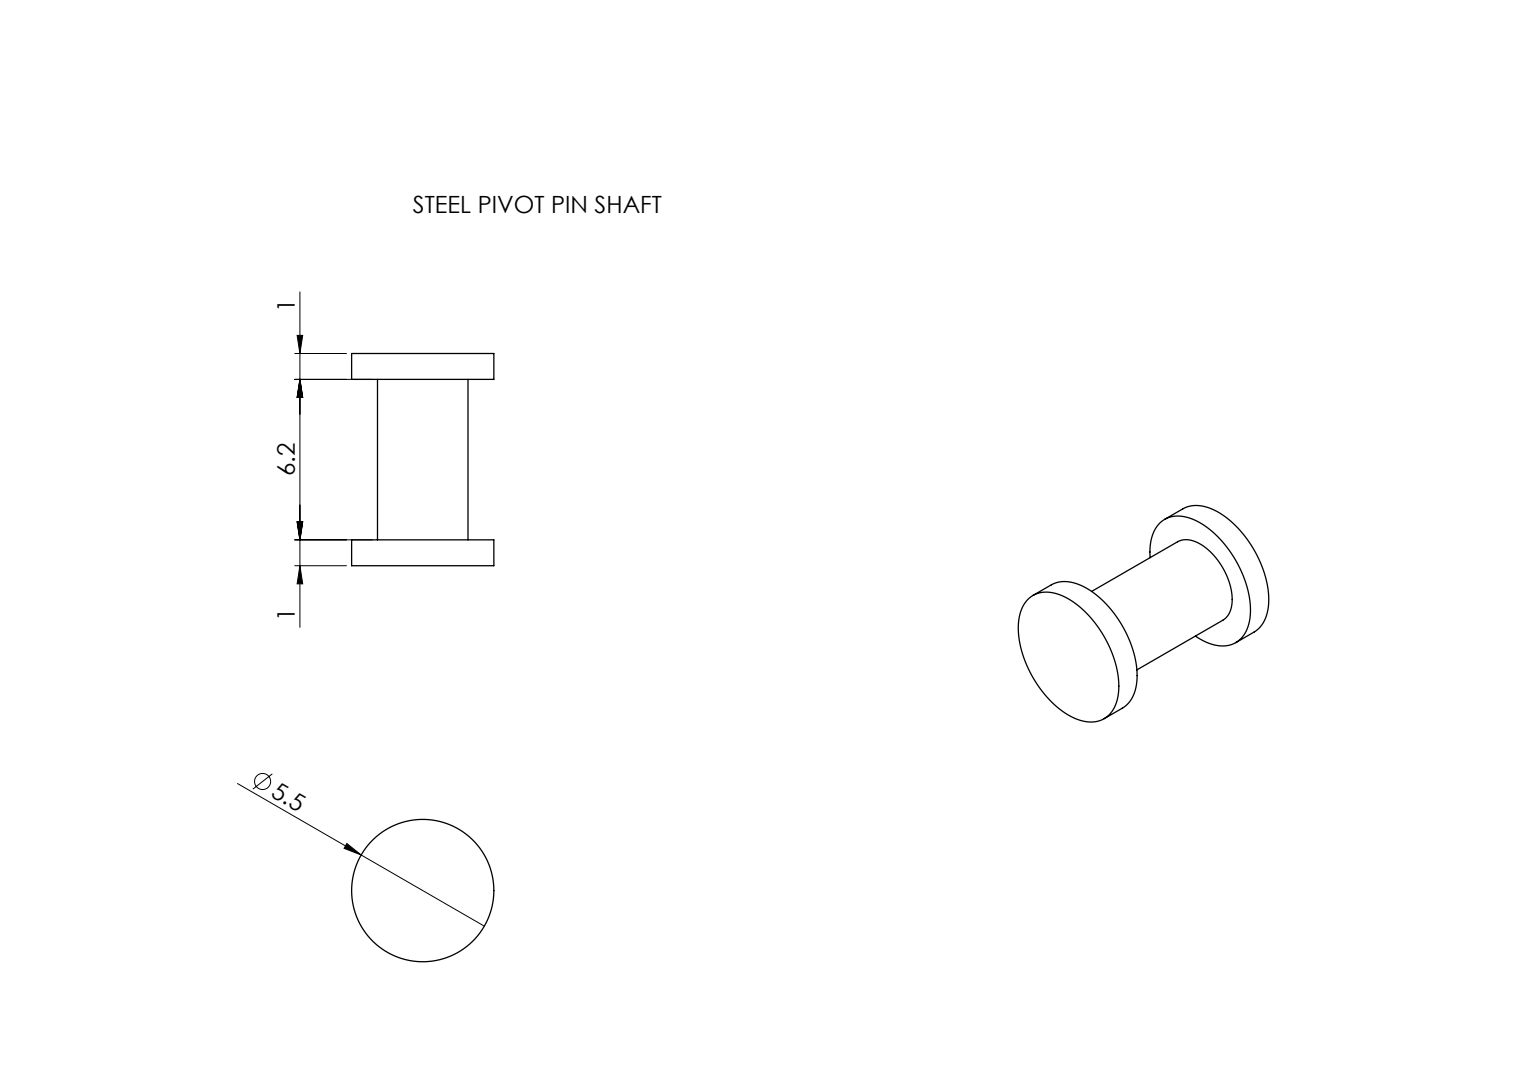
ISO-10303-21;
HEADER;
FILE_DESCRIPTION (('STEP AP214'),
    '1' );
FILE_NAME ('Steel Pivot Pin Shaft.step',
    '2026-09-30T04:43:20',
    ( '' ),
    ( '' ),
    'SwSTEP 2.0',
    'SolidWorks 2026',
    '' );
FILE_SCHEMA (( 'AUTOMOTIVE_DESIGN' ));
ENDSEC;

DATA;
#339=EDGE_CURVE ( 'NONE', #23586, #15428, #53300, .T. ) ;
#351=CARTESIAN_POINT ( 'NONE',  ( -6.110905869600904872, 1.712176620043476140E-14, 3.600000000000000089 ) ) ;
#366=EDGE_LOOP ( 'NONE', ( #1218, #51641 ) ) ;
#396=ORIENTED_EDGE ( 'NONE', *, *, #51721, .F. ) ;
#484=DIRECTION ( 'NONE',  ( 0.000000000000000000, 0.000000000000000000, 1.000000000000000000 ) ) ;
#1065=DIRECTION ( 'NONE',  ( 0.000000000000000000, 0.000000000000000000, -1.000000000000000000 ) ) ;
#1143=ORIENTED_EDGE ( 'NONE', *, *, #9429, .T. ) ;
#1218=ORIENTED_EDGE ( 'NONE', *, *, #16405, .T. ) ;
#1370=EDGE_LOOP ( 'NONE', ( #41531, #53817 ) ) ;
#1691=AXIS2_PLACEMENT_3D ( 'NONE', #351, #44090, #52871 ) ;
#1703=CARTESIAN_POINT ( 'NONE',  ( -6.110905869600904872, 1.712176620043476140E-14, -3.600000000000000089 ) ) ;
#1760=( GEOMETRIC_REPRESENTATION_CONTEXT ( 3 ) GLOBAL_UNCERTAINTY_ASSIGNED_CONTEXT ( ( #42179 ) ) GLOBAL_UNIT_ASSIGNED_CONTEXT ( ( #39762, #23813, #2772 ) ) REPRESENTATION_CONTEXT ( 'NONE', 'WORKASPACE' ) );
#1875=VERTEX_POINT ( 'NONE', #20074 ) ;
#1894=EDGE_LOOP ( 'NONE', ( #21734, #23060 ) ) ;
#2067=EDGE_LOOP ( 'NONE', ( #37855, #52540, #10327, #27541 ) ) ;
#2068=DIRECTION ( 'NONE',  ( -1.000000000000000000, 0.000000000000000000, 0.000000000000000000 ) ) ;
#2078=AXIS2_PLACEMENT_3D ( 'NONE', #1703, #6268, #15329 ) ;
#2169=EDGE_CURVE ( 'NONE', #13325, #33916, #33726, .T. ) ;
#2253=VECTOR ( 'NONE', #43903, 1000.000000000000000 ) ;
#2401=CARTESIAN_POINT ( 'NONE',  ( -6.110905869600904872, 1.712176620043476140E-14, 2.600000000000000089 ) ) ;
#2458=FACE_OUTER_BOUND ( 'NONE', #1370, .T. ) ;
#2610=AXIS2_PLACEMENT_3D ( 'NONE', #34638, #13373, #3697 ) ;
#2772=( NAMED_UNIT ( * ) SI_UNIT ( $, .STERADIAN. ) SOLID_ANGLE_UNIT ( ) );
#3052=CARTESIAN_POINT ( 'NONE',  ( -3.360905869600907092, 1.745854407020028306E-14, 3.600000000000000089 ) ) ;
#3156=SHAPE_REPRESENTATION ( 'Steel Pivot Pin Shaft', ( #2610 ), #1760 ) ;
#3558=UNCERTAINTY_MEASURE_WITH_UNIT (LENGTH_MEASURE( 1.000000000000000082E-05 ), #11031, 'distance_accuracy_value', 'NONE');
#3697=DIRECTION ( 'NONE',  ( 1.000000000000000000, 0.000000000000000000, 0.000000000000000000 ) ) ;
#3719=ADVANCED_FACE ( 'NONE', ( #23132 ), #6367, .T. ) ;
#4027=AXIS2_PLACEMENT_3D ( 'NONE', #41047, #46142, #45878 ) ;
#4059=CIRCLE ( 'NONE', #6771, 2.749999999999997335 ) ;
#4638=DIRECTION ( 'NONE',  ( -1.000000000000000000, 0.000000000000000000, 0.000000000000000000 ) ) ;
#5017=ORIENTED_EDGE ( 'NONE', *, *, #54598, .F. ) ;
#5743=APPLICATION_CONTEXT ( 'automotive_design' ) ;
#5928=AXIS2_PLACEMENT_3D ( 'NONE', #44296, #53097, #40307 ) ;
#6268=DIRECTION ( 'NONE',  ( 0.000000000000000000, 0.000000000000000000, -1.000000000000000000 ) ) ;
#6367=CYLINDRICAL_SURFACE ( 'NONE', #37649, 1.750000000000003331 ) ;
#6536=AXIS2_PLACEMENT_3D ( 'NONE', #26903, #484, #8748 ) ;
#6615=VERTEX_POINT ( 'NONE', #41477 ) ;
#6732=EDGE_CURVE ( 'NONE', #6615, #10587, #21831, .T. ) ;
#6771=AXIS2_PLACEMENT_3D ( 'NONE', #23374, #27624, #40690 ) ;
#6831=CLOSED_SHELL ( 'NONE', ( #47988, #39827, #3719, #23415, #26829, #43131, #39539, #24833, #28152, #23876 ) ) ;
#6962=DIRECTION ( 'NONE',  ( 0.000000000000000000, 0.000000000000000000, 1.000000000000000000 ) ) ;
#6987=VERTEX_POINT ( 'NONE', #32867 ) ;
#7083=FILL_AREA_STYLE_COLOUR ( '', #10850 ) ;
#7134=CARTESIAN_POINT ( 'NONE',  ( -3.360905869600907092, 1.712176620043476140E-14, -3.600000000000000089 ) ) ;
#7765=CARTESIAN_POINT ( 'NONE',  ( -8.860905869600903983, 1.712176620043476140E-14, 3.600000000000000089 ) ) ;
#7964=DIRECTION ( 'NONE',  ( -0.000000000000000000, -0.000000000000000000, 1.000000000000000000 ) ) ;
#8573=VECTOR ( 'NONE', #42169, 1000.000000000000000 ) ;
#8748=DIRECTION ( 'NONE',  ( 1.000000000000000000, 0.000000000000000000, 0.000000000000000000 ) ) ;
#9041=CARTESIAN_POINT ( 'NONE',  ( -4.360905869600901319, 1.733607939028554791E-14, -3.600000000000000089 ) ) ;
#9135=ORIENTED_EDGE ( 'NONE', *, *, #55863, .F. ) ;
#9429=EDGE_CURVE ( 'NONE', #6987, #33042, #15488, .T. ) ;
#9446=CARTESIAN_POINT ( 'NONE',  ( -6.110905869600904872, 1.712176620043476140E-14, 2.600000000000000089 ) ) ;
#9702=CYLINDRICAL_SURFACE ( 'NONE', #40281, 2.749999999999997780 ) ;
#9786=ORIENTED_EDGE ( 'NONE', *, *, #25713, .F. ) ;
#10212=AXIS2_PLACEMENT_3D ( 'NONE', #50763, #55050, #45962 ) ;
#10236=DIRECTION ( 'NONE',  ( 1.000000000000000000, 0.000000000000000000, 0.000000000000000000 ) ) ;
#10327=ORIENTED_EDGE ( 'NONE', *, *, #54598, .T. ) ;
#10570=FILL_AREA_STYLE_COLOUR ( '', #28482 ) ;
#10587=VERTEX_POINT ( 'NONE', #20963 ) ;
#10850=COLOUR_RGB ( '', 0.72549020, 0.75294118, 0.79215686) ;
#11031=( LENGTH_UNIT ( ) NAMED_UNIT ( * ) SI_UNIT ( .MILLI., .METRE. ) );
#11661=FILL_AREA_STYLE ('',( #10570 ) ) ;
#11865=SURFACE_STYLE_USAGE ( .BOTH. , #32620 ) ;
#12149=MECHANICAL_DESIGN_GEOMETRIC_PRESENTATION_REPRESENTATION('',(#43002),#55684);
#12473=DIRECTION ( 'NONE',  ( 0.000000000000000000, 0.000000000000000000, 1.000000000000000000 ) ) ;
#12683=MECHANICAL_DESIGN_GEOMETRIC_PRESENTATION_REPRESENTATION('',(#46182),#19000);
#13325=VERTEX_POINT ( 'NONE', #15566 ) ;
#13373=DIRECTION ( 'NONE',  ( 0.000000000000000000, 0.000000000000000000, 1.000000000000000000 ) ) ;
#13649=DIRECTION ( 'NONE',  ( -0.000000000000000000, -0.000000000000000000, 1.000000000000000000 ) ) ;
#13919=ORIENTED_EDGE ( 'NONE', *, *, #51721, .T. ) ;
#14396=CARTESIAN_POINT ( 'NONE',  ( -3.360905869600907092, 1.712176620043476140E-14, -4.599999999999999645 ) ) ;
#14547=DIRECTION ( 'NONE',  ( 0.000000000000000000, 0.000000000000000000, 1.000000000000000000 ) ) ;
#14842=AXIS2_PLACEMENT_3D ( 'NONE', #40048, #27012, #10236 ) ;
#14859=EDGE_LOOP ( 'NONE', ( #20763, #21521, #39292, #31255 ) ) ;
#15099=SURFACE_STYLE_USAGE ( .BOTH. , #45722 ) ;
#15329=DIRECTION ( 'NONE',  ( -1.000000000000000000, 0.000000000000000000, -0.000000000000000000 ) ) ;
#15428=VERTEX_POINT ( 'NONE', #7134 ) ;
#15488=CIRCLE ( 'NONE', #46317, 1.750000000000003331 ) ;
#15566=CARTESIAN_POINT ( 'NONE',  ( -8.860905869600903983, 1.712176620043476140E-14, 3.600000000000000089 ) ) ;
#16398=EDGE_CURVE ( 'NONE', #33916, #43669, #20608, .T. ) ;
#16405=EDGE_CURVE ( 'NONE', #53889, #44242, #24860, .T. ) ;
#16724=ORIENTED_EDGE ( 'NONE', *, *, #9429, .F. ) ;
#17002=EDGE_LOOP ( 'NONE', ( #45520, #34695 ) ) ;
#17694=PLANE ( 'NONE',  #33826 ) ;
#17939=FACE_OUTER_BOUND ( 'NONE', #14859, .T. ) ;
#18204=EDGE_CURVE ( 'NONE', #33042, #6987, #54958, .T. ) ;
#18215=CARTESIAN_POINT ( 'NONE',  ( -6.110905869600904872, 1.712176620043476140E-14, -3.600000000000000089 ) ) ;
#18260=PRODUCT_DEFINITION_SHAPE ( 'NONE', 'NONE',  #35061 ) ;
#18382=AXIS2_PLACEMENT_3D ( 'NONE', #24725, #33816, #29581 ) ;
#18499=AXIS2_PLACEMENT_3D ( 'NONE', #49858, #28274, #37345 ) ;
#18809=DIRECTION ( 'NONE',  ( 0.000000000000000000, 0.000000000000000000, 1.000000000000000000 ) ) ;
#19000=( GEOMETRIC_REPRESENTATION_CONTEXT ( 3 ) GLOBAL_UNCERTAINTY_ASSIGNED_CONTEXT ( ( #3558 ) ) GLOBAL_UNIT_ASSIGNED_CONTEXT ( ( #11031, #40863, #33466 ) ) REPRESENTATION_CONTEXT ( 'NONE', 'WORKASPACE' ) );
#19278=CARTESIAN_POINT ( 'NONE',  ( -4.360905869600901319, 1.733607939028554791E-14, 2.600000000000000089 ) ) ;
#19415=CARTESIAN_POINT ( 'NONE',  ( -4.360905869600901319, 1.733607939028554791E-14, 2.600000000000000089 ) ) ;
#19808=CIRCLE ( 'NONE', #1691, 2.749999999999998224 ) ;
#19916=PRODUCT_DEFINITION_FORMATION_WITH_SPECIFIED_SOURCE ( 'ANY', '', #27850, .NOT_KNOWN. ) ;
#20074=CARTESIAN_POINT ( 'NONE',  ( -8.860905869600903983, 1.712176620043476140E-14, 2.600000000000000089 ) ) ;
#20081=AXIS2_PLACEMENT_3D ( 'NONE', #48959, #44994, #2068 ) ;
#20150=PRESENTATION_STYLE_ASSIGNMENT (( #15099 ) ) ;
#20201=CIRCLE ( 'NONE', #10212, 2.749999999999998224 ) ;
#20608=LINE ( 'NONE', #28264, #8573 ) ;
#20695=SHAPE_DEFINITION_REPRESENTATION ( #18260, #3156 ) ;
#20763=ORIENTED_EDGE ( 'NONE', *, *, #6732, .F. ) ;
#20963=CARTESIAN_POINT ( 'NONE',  ( -8.860905869600902207, 1.745854407020028306E-14, -3.600000000000000089 ) ) ;
#21107=CARTESIAN_POINT ( 'NONE',  ( -6.110905869600904872, 1.712176620043476140E-14, -4.599999999999999645 ) ) ;
#21394=ORIENTED_EDGE ( 'NONE', *, *, #16405, .F. ) ;
#21478=EDGE_CURVE ( 'NONE', #1875, #43669, #20201, .T. ) ;
#21521=ORIENTED_EDGE ( 'NONE', *, *, #42925, .F. ) ;
#21734=ORIENTED_EDGE ( 'NONE', *, *, #2169, .T. ) ;
#21831=LINE ( 'NONE', #46855, #54507 ) ;
#21855=DIRECTION ( 'NONE',  ( -1.000000000000000000, 0.000000000000000000, 0.000000000000000000 ) ) ;
#22356=DIRECTION ( 'NONE',  ( -0.000000000000000000, -0.000000000000000000, 1.000000000000000000 ) ) ;
#22763=DIRECTION ( 'NONE',  ( 1.000000000000000000, 0.000000000000000000, 0.000000000000000000 ) ) ;
#23060=ORIENTED_EDGE ( 'NONE', *, *, #55863, .T. ) ;
#23072=FACE_OUTER_BOUND ( 'NONE', #17002, .T. ) ;
#23132=FACE_OUTER_BOUND ( 'NONE', #53242, .T. ) ;
#23250=DIRECTION ( 'NONE',  ( -1.000000000000000000, 0.000000000000000000, 0.000000000000000000 ) ) ;
#23374=CARTESIAN_POINT ( 'NONE',  ( -6.110905869600904872, 1.712176620043476140E-14, -3.600000000000000089 ) ) ;
#23415=ADVANCED_FACE ( 'NONE', ( #43809 ), #34738, .T. ) ;
#23458=ORIENTED_EDGE ( 'NONE', *, *, #6732, .T. ) ;
#23586=VERTEX_POINT ( 'NONE', #42905 ) ;
#23813=( NAMED_UNIT ( * ) PLANE_ANGLE_UNIT ( ) SI_UNIT ( $, .RADIAN. ) );
#23837=FACE_OUTER_BOUND ( 'NONE', #51240, .T. ) ;
#23876=ADVANCED_FACE ( 'NONE', ( #27550, #23837 ), #49947, .F. ) ;
#24166=AXIS2_PLACEMENT_3D ( 'NONE', #53600, #1065, #23250 ) ;
#24573=DIRECTION ( 'NONE',  ( 0.000000000000000000, 0.000000000000000000, -1.000000000000000000 ) ) ;
#24725=CARTESIAN_POINT ( 'NONE',  ( -6.110905869600904872, 1.712176620043476140E-14, 3.600000000000000089 ) ) ;
#24833=ADVANCED_FACE ( 'NONE', ( #17939 ), #9702, .T. ) ;
#24860=CIRCLE ( 'NONE', #4027, 1.750000000000003331 ) ;
#25713=EDGE_CURVE ( 'NONE', #53889, #6987, #43073, .T. ) ;
#26591=ADVANCED_BREP_SHAPE_REPRESENTATION ( '', ( #41703, #2610 ), #1760 ) ;
#26774=ORIENTED_EDGE ( 'NONE', *, *, #37370, .T. ) ;
#26829=ADVANCED_FACE ( 'NONE', ( #40983 ), #35923, .T. ) ;
#26903=CARTESIAN_POINT ( 'NONE',  ( -6.110905869600904872, 1.712176620043476140E-14, 3.600000000000000089 ) ) ;
#27012=DIRECTION ( 'NONE',  ( -0.000000000000000000, -0.000000000000000000, 1.000000000000000000 ) ) ;
#27541=ORIENTED_EDGE ( 'NONE', *, *, #21478, .T. ) ;
#27550=FACE_BOUND ( 'NONE', #39735, .T. ) ;
#27624=DIRECTION ( 'NONE',  ( 0.000000000000000000, 0.000000000000000000, -1.000000000000000000 ) ) ;
#27850=PRODUCT ( 'Steel Pivot Pin Shaft', 'Steel Pivot Pin Shaft', '', ( #47354 ) ) ;
#28152=ADVANCED_FACE ( 'NONE', ( #2458 ), #53847, .T. ) ;
#28264=CARTESIAN_POINT ( 'NONE',  ( -3.360905869600907092, 1.745854407020028306E-14, 3.600000000000000089 ) ) ;
#28274=DIRECTION ( 'NONE',  ( 0.000000000000000000, 0.000000000000000000, 1.000000000000000000 ) ) ;
#28349=SURFACE_STYLE_FILL_AREA ( #55061 ) ;
#28482=COLOUR_RGB ( '', 0.72549020, 0.75294118, 0.79215686) ;
#28514=DIRECTION ( 'NONE',  ( 1.000000000000000000, 0.000000000000000000, 0.000000000000000000 ) ) ;
#28840=ORIENTED_EDGE ( 'NONE', *, *, #18204, .T. ) ;
#28864=CARTESIAN_POINT ( 'NONE',  ( -6.110905869600904872, 1.712176620043476140E-14, -4.599999999999999645 ) ) ;
#28976=SURFACE_STYLE_FILL_AREA ( #11661 ) ;
#29581=DIRECTION ( 'NONE',  ( -1.000000000000000000, 0.000000000000000000, 0.000000000000000000 ) ) ;
#29710=PRODUCT_DEFINITION_CONTEXT ( 'detailed design', #32927, 'design' ) ;
#29750=ORIENTED_EDGE ( 'NONE', *, *, #49770, .F. ) ;
#30226=EDGE_LOOP ( 'NONE', ( #40736, #23458, #13919, #53598 ) ) ;
#30368=AXIS2_PLACEMENT_3D ( 'NONE', #34632, #34944, #21855 ) ;
#30388=VECTOR ( 'NONE', #22356, 1000.000000000000000 ) ;
#30508=DIRECTION ( 'NONE',  ( -0.000000000000000000, -0.000000000000000000, -1.000000000000000000 ) ) ;
#30616=CARTESIAN_POINT ( 'NONE',  ( -7.860905869600908424, 1.712176620043476140E-14, 2.600000000000000089 ) ) ;
#31255=ORIENTED_EDGE ( 'NONE', *, *, #49770, .T. ) ;
#31440=CIRCLE ( 'NONE', #24166, 2.749999999999997335 ) ;
#31939=AXIS2_PLACEMENT_3D ( 'NONE', #2401, #6962, #28514 ) ;
#32620=SURFACE_SIDE_STYLE ('',( #28349 ) ) ;
#32867=CARTESIAN_POINT ( 'NONE',  ( -7.860905869600908424, 1.712176620043476140E-14, -3.600000000000000089 ) ) ;
#32927=APPLICATION_CONTEXT ( 'automotive_design' ) ;
#33042=VERTEX_POINT ( 'NONE', #9041 ) ;
#33069=EDGE_LOOP ( 'NONE', ( #33318, #21394, #33430, #1143 ) ) ;
#33318=ORIENTED_EDGE ( 'NONE', *, *, #37370, .F. ) ;
#33430=ORIENTED_EDGE ( 'NONE', *, *, #25713, .T. ) ;
#33466=( NAMED_UNIT ( * ) SI_UNIT ( $, .STERADIAN. ) SOLID_ANGLE_UNIT ( ) );
#33726=CIRCLE ( 'NONE', #6536, 2.749999999999998224 ) ;
#33816=DIRECTION ( 'NONE',  ( -0.000000000000000000, -0.000000000000000000, -1.000000000000000000 ) ) ;
#33826=AXIS2_PLACEMENT_3D ( 'NONE', #9446, #14547, #35866 ) ;
#33916=VERTEX_POINT ( 'NONE', #3052 ) ;
#34433=DIRECTION ( 'NONE',  ( -0.000000000000000000, -0.000000000000000000, -1.000000000000000000 ) ) ;
#34541=CARTESIAN_POINT ( 'NONE',  ( -7.860905869600908424, 1.712176620043476140E-14, 2.600000000000000089 ) ) ;
#34632=CARTESIAN_POINT ( 'NONE',  ( -6.110905869600904872, 1.712176620043476140E-14, -4.599999999999999645 ) ) ;
#34638=CARTESIAN_POINT ( 'NONE',  ( 0.000000000000000000, 0.000000000000000000, 0.000000000000000000 ) ) ;
#34695=ORIENTED_EDGE ( 'NONE', *, *, #36075, .F. ) ;
#34738=CYLINDRICAL_SURFACE ( 'NONE', #50074, 1.750000000000003331 ) ;
#34944=DIRECTION ( 'NONE',  ( 0.000000000000000000, 0.000000000000000000, -1.000000000000000000 ) ) ;
#35061=PRODUCT_DEFINITION ( 'UNKNOWN', '', #19916, #29710 ) ;
#35480=PLANE ( 'NONE',  #5928 ) ;
#35512=CYLINDRICAL_SURFACE ( 'NONE', #14842, 2.749999999999997780 ) ;
#35814=DIRECTION ( 'NONE',  ( 1.000000000000000000, 0.000000000000000000, 0.000000000000000000 ) ) ;
#35866=DIRECTION ( 'NONE',  ( 1.000000000000000000, 0.000000000000000000, -0.000000000000000000 ) ) ;
#35923=CYLINDRICAL_SURFACE ( 'NONE', #20081, 2.749999999999999112 ) ;
#36075=EDGE_CURVE ( 'NONE', #43669, #1875, #39391, .T. ) ;
#36732=CIRCLE ( 'NONE', #45752, 2.749999999999997335 ) ;
#37207=( NAMED_UNIT ( * ) PLANE_ANGLE_UNIT ( ) SI_UNIT ( $, .RADIAN. ) );
#37345=DIRECTION ( 'NONE',  ( 1.000000000000000000, 0.000000000000000000, 0.000000000000000000 ) ) ;
#37370=EDGE_CURVE ( 'NONE', #44242, #33042, #49240, .T. ) ;
#37649=AXIS2_PLACEMENT_3D ( 'NONE', #40732, #40462, #41282 ) ;
#37739=SHAPE_REPRESENTATION_RELATIONSHIP ( 'NONE' , 'NONE' ,  #3156, #26591 ) ;
#37855=ORIENTED_EDGE ( 'NONE', *, *, #16398, .F. ) ;
#38546=CIRCLE ( 'NONE', #30368, 2.749999999999997335 ) ;
#38576=VECTOR ( 'NONE', #54075, 1000.000000000000000 ) ;
#39292=ORIENTED_EDGE ( 'NONE', *, *, #339, .T. ) ;
#39391=CIRCLE ( 'NONE', #18499, 2.749999999999998224 ) ;
#39539=ADVANCED_FACE ( 'NONE', ( #53190, #23072 ), #17694, .F. ) ;
#39735=EDGE_LOOP ( 'NONE', ( #16724, #43130 ) ) ;
#39762=( LENGTH_UNIT ( ) NAMED_UNIT ( * ) SI_UNIT ( .MILLI., .METRE. ) );
#39827=ADVANCED_FACE ( 'NONE', ( #42893 ), #46298, .T. ) ;
#40015=FACE_OUTER_BOUND ( 'NONE', #1894, .T. ) ;
#40048=CARTESIAN_POINT ( 'NONE',  ( -6.110905869600904872, 1.712176620043476140E-14, -4.599999999999999645 ) ) ;
#40281=AXIS2_PLACEMENT_3D ( 'NONE', #51990, #13649, #35814 ) ;
#40307=DIRECTION ( 'NONE',  ( 1.000000000000000000, 0.000000000000000000, -0.000000000000000000 ) ) ;
#40462=DIRECTION ( 'NONE',  ( -0.000000000000000000, -0.000000000000000000, -1.000000000000000000 ) ) ;
#40690=DIRECTION ( 'NONE',  ( -1.000000000000000000, 0.000000000000000000, 0.000000000000000000 ) ) ;
#40732=CARTESIAN_POINT ( 'NONE',  ( -6.110905869600904872, 1.712176620043476140E-14, 2.600000000000000089 ) ) ;
#40736=ORIENTED_EDGE ( 'NONE', *, *, #49477, .F. ) ;
#40863=( NAMED_UNIT ( * ) PLANE_ANGLE_UNIT ( ) SI_UNIT ( $, .RADIAN. ) );
#40983=FACE_OUTER_BOUND ( 'NONE', #2067, .T. ) ;
#41047=CARTESIAN_POINT ( 'NONE',  ( -6.110905869600904872, 1.712176620043476140E-14, 2.600000000000000089 ) ) ;
#41282=DIRECTION ( 'NONE',  ( -1.000000000000000000, 0.000000000000000000, 0.000000000000000000 ) ) ;
#41477=CARTESIAN_POINT ( 'NONE',  ( -8.860905869600902207, 1.745854407020028306E-14, -4.599999999999999645 ) ) ;
#41531=ORIENTED_EDGE ( 'NONE', *, *, #42925, .T. ) ;
#41703=MANIFOLD_SOLID_BREP ( 'Boss-Extrude3', #6831 ) ;
#41821=ORIENTED_EDGE ( 'NONE', *, *, #16398, .T. ) ;
#41967=CARTESIAN_POINT ( 'NONE',  ( -6.110905869600904872, 1.712176620043476140E-14, -3.600000000000000089 ) ) ;
#42023=( NAMED_UNIT ( * ) SI_UNIT ( $, .STERADIAN. ) SOLID_ANGLE_UNIT ( ) );
#42169=DIRECTION ( 'NONE',  ( -0.000000000000000000, -0.000000000000000000, -1.000000000000000000 ) ) ;
#42179=UNCERTAINTY_MEASURE_WITH_UNIT (LENGTH_MEASURE( 1.000000000000000082E-05 ), #39762, 'distance_accuracy_value', 'NONE');
#42893=FACE_OUTER_BOUND ( 'NONE', #50812, .T. ) ;
#42905=CARTESIAN_POINT ( 'NONE',  ( -3.360905869600907092, 1.712176620043476140E-14, -4.599999999999999645 ) ) ;
#42925=EDGE_CURVE ( 'NONE', #23586, #6615, #38546, .T. ) ;
#42951=LINE ( 'NONE', #7765, #48780 ) ;
#43002=STYLED_ITEM ( 'NONE', ( #20150 ), #41703 ) ;
#43073=LINE ( 'NONE', #34541, #2253 ) ;
#43130=ORIENTED_EDGE ( 'NONE', *, *, #18204, .F. ) ;
#43131=ADVANCED_FACE ( 'NONE', ( #40015 ), #35480, .T. ) ;
#43669=VERTEX_POINT ( 'NONE', #54990 ) ;
#43809=FACE_OUTER_BOUND ( 'NONE', #33069, .T. ) ;
#43903=DIRECTION ( 'NONE',  ( -0.000000000000000000, -0.000000000000000000, -1.000000000000000000 ) ) ;
#44090=DIRECTION ( 'NONE',  ( 0.000000000000000000, 0.000000000000000000, 1.000000000000000000 ) ) ;
#44242=VERTEX_POINT ( 'NONE', #19278 ) ;
#44296=CARTESIAN_POINT ( 'NONE',  ( -6.110905869600904872, 1.712176620043476140E-14, 3.600000000000000089 ) ) ;
#44994=DIRECTION ( 'NONE',  ( -0.000000000000000000, -0.000000000000000000, -1.000000000000000000 ) ) ;
#45520=ORIENTED_EDGE ( 'NONE', *, *, #21478, .F. ) ;
#45722=SURFACE_SIDE_STYLE ('',( #28976 ) ) ;
#45752=AXIS2_PLACEMENT_3D ( 'NONE', #21107, #55465, #46117 ) ;
#45878=DIRECTION ( 'NONE',  ( 1.000000000000000000, 0.000000000000000000, 0.000000000000000000 ) ) ;
#45962=DIRECTION ( 'NONE',  ( 1.000000000000000000, 0.000000000000000000, 0.000000000000000000 ) ) ;
#46117=DIRECTION ( 'NONE',  ( -1.000000000000000000, 0.000000000000000000, 0.000000000000000000 ) ) ;
#46142=DIRECTION ( 'NONE',  ( 0.000000000000000000, 0.000000000000000000, 1.000000000000000000 ) ) ;
#46174=EDGE_CURVE ( 'NONE', #44242, #53889, #48255, .T. ) ;
#46182=STYLED_ITEM ( 'NONE', ( #49924 ), #26591 ) ;
#46273=( LENGTH_UNIT ( ) NAMED_UNIT ( * ) SI_UNIT ( .MILLI., .METRE. ) );
#46298=CYLINDRICAL_SURFACE ( 'NONE', #18382, 2.749999999999999112 ) ;
#46317=AXIS2_PLACEMENT_3D ( 'NONE', #41967, #12473, #55066 ) ;
#46471=AXIS2_PLACEMENT_3D ( 'NONE', #28864, #24573, #49318 ) ;
#46763=AXIS2_PLACEMENT_3D ( 'NONE', #18215, #18809, #22763 ) ;
#46855=CARTESIAN_POINT ( 'NONE',  ( -8.860905869600902207, 1.745854407020028306E-14, -4.599999999999999645 ) ) ;
#47354=PRODUCT_CONTEXT ( 'NONE', #5743, 'mechanical' ) ;
#47443=ORIENTED_EDGE ( 'NONE', *, *, #36075, .T. ) ;
#47988=ADVANCED_FACE ( 'NONE', ( #49421 ), #35512, .T. ) ;
#48255=CIRCLE ( 'NONE', #31939, 1.750000000000003331 ) ;
#48780=VECTOR ( 'NONE', #34433, 1000.000000000000000 ) ;
#48959=CARTESIAN_POINT ( 'NONE',  ( -6.110905869600904872, 1.712176620043476140E-14, 3.600000000000000089 ) ) ;
#49240=LINE ( 'NONE', #19415, #38576 ) ;
#49318=DIRECTION ( 'NONE',  ( -1.000000000000000000, 0.000000000000000000, -0.000000000000000000 ) ) ;
#49421=FACE_OUTER_BOUND ( 'NONE', #30226, .T. ) ;
#49477=EDGE_CURVE ( 'NONE', #6615, #23586, #36732, .T. ) ;
#49770=EDGE_CURVE ( 'NONE', #15428, #10587, #4059, .T. ) ;
#49858=CARTESIAN_POINT ( 'NONE',  ( -6.110905869600904872, 1.712176620043476140E-14, 2.600000000000000089 ) ) ;
#49924=PRESENTATION_STYLE_ASSIGNMENT (( #11865 ) ) ;
#49947=PLANE ( 'NONE',  #2078 ) ;
#50074=AXIS2_PLACEMENT_3D ( 'NONE', #52055, #30508, #4638 ) ;
#50763=CARTESIAN_POINT ( 'NONE',  ( -6.110905869600904872, 1.712176620043476140E-14, 2.600000000000000089 ) ) ;
#50812=EDGE_LOOP ( 'NONE', ( #9135, #41821, #47443, #5017 ) ) ;
#51240=EDGE_LOOP ( 'NONE', ( #29750, #396 ) ) ;
#51641=ORIENTED_EDGE ( 'NONE', *, *, #46174, .T. ) ;
#51721=EDGE_CURVE ( 'NONE', #10587, #15428, #31440, .T. ) ;
#51990=CARTESIAN_POINT ( 'NONE',  ( -6.110905869600904872, 1.712176620043476140E-14, -4.599999999999999645 ) ) ;
#52055=CARTESIAN_POINT ( 'NONE',  ( -6.110905869600904872, 1.712176620043476140E-14, 2.600000000000000089 ) ) ;
#52540=ORIENTED_EDGE ( 'NONE', *, *, #2169, .F. ) ;
#52871=DIRECTION ( 'NONE',  ( 1.000000000000000000, 0.000000000000000000, 0.000000000000000000 ) ) ;
#53097=DIRECTION ( 'NONE',  ( 0.000000000000000000, 0.000000000000000000, 1.000000000000000000 ) ) ;
#53190=FACE_BOUND ( 'NONE', #366, .T. ) ;
#53242=EDGE_LOOP ( 'NONE', ( #55877, #26774, #28840, #9786 ) ) ;
#53300=LINE ( 'NONE', #14396, #30388 ) ;
#53598=ORIENTED_EDGE ( 'NONE', *, *, #339, .F. ) ;
#53600=CARTESIAN_POINT ( 'NONE',  ( -6.110905869600904872, 1.712176620043476140E-14, -3.600000000000000089 ) ) ;
#53817=ORIENTED_EDGE ( 'NONE', *, *, #49477, .T. ) ;
#53847=PLANE ( 'NONE',  #46471 ) ;
#53889=VERTEX_POINT ( 'NONE', #30616 ) ;
#54075=DIRECTION ( 'NONE',  ( -0.000000000000000000, -0.000000000000000000, -1.000000000000000000 ) ) ;
#54507=VECTOR ( 'NONE', #7964, 1000.000000000000000 ) ;
#54598=EDGE_CURVE ( 'NONE', #13325, #1875, #42951, .T. ) ;
#54661=UNCERTAINTY_MEASURE_WITH_UNIT (LENGTH_MEASURE( 1.000000000000000082E-05 ), #46273, 'distance_accuracy_value', 'NONE');
#54958=CIRCLE ( 'NONE', #46763, 1.750000000000003331 ) ;
#54990=CARTESIAN_POINT ( 'NONE',  ( -3.360905869600907092, 1.745854407020028306E-14, 2.600000000000000089 ) ) ;
#55050=DIRECTION ( 'NONE',  ( 0.000000000000000000, 0.000000000000000000, 1.000000000000000000 ) ) ;
#55061=FILL_AREA_STYLE ('',( #7083 ) ) ;
#55066=DIRECTION ( 'NONE',  ( 1.000000000000000000, 0.000000000000000000, 0.000000000000000000 ) ) ;
#55465=DIRECTION ( 'NONE',  ( 0.000000000000000000, 0.000000000000000000, -1.000000000000000000 ) ) ;
#55684=( GEOMETRIC_REPRESENTATION_CONTEXT ( 3 ) GLOBAL_UNCERTAINTY_ASSIGNED_CONTEXT ( ( #54661 ) ) GLOBAL_UNIT_ASSIGNED_CONTEXT ( ( #46273, #37207, #42023 ) ) REPRESENTATION_CONTEXT ( 'NONE', 'WORKASPACE' ) );
#55863=EDGE_CURVE ( 'NONE', #33916, #13325, #19808, .T. ) ;
#55877=ORIENTED_EDGE ( 'NONE', *, *, #46174, .F. ) ;
ENDSEC;
END-ISO-10303-21;
